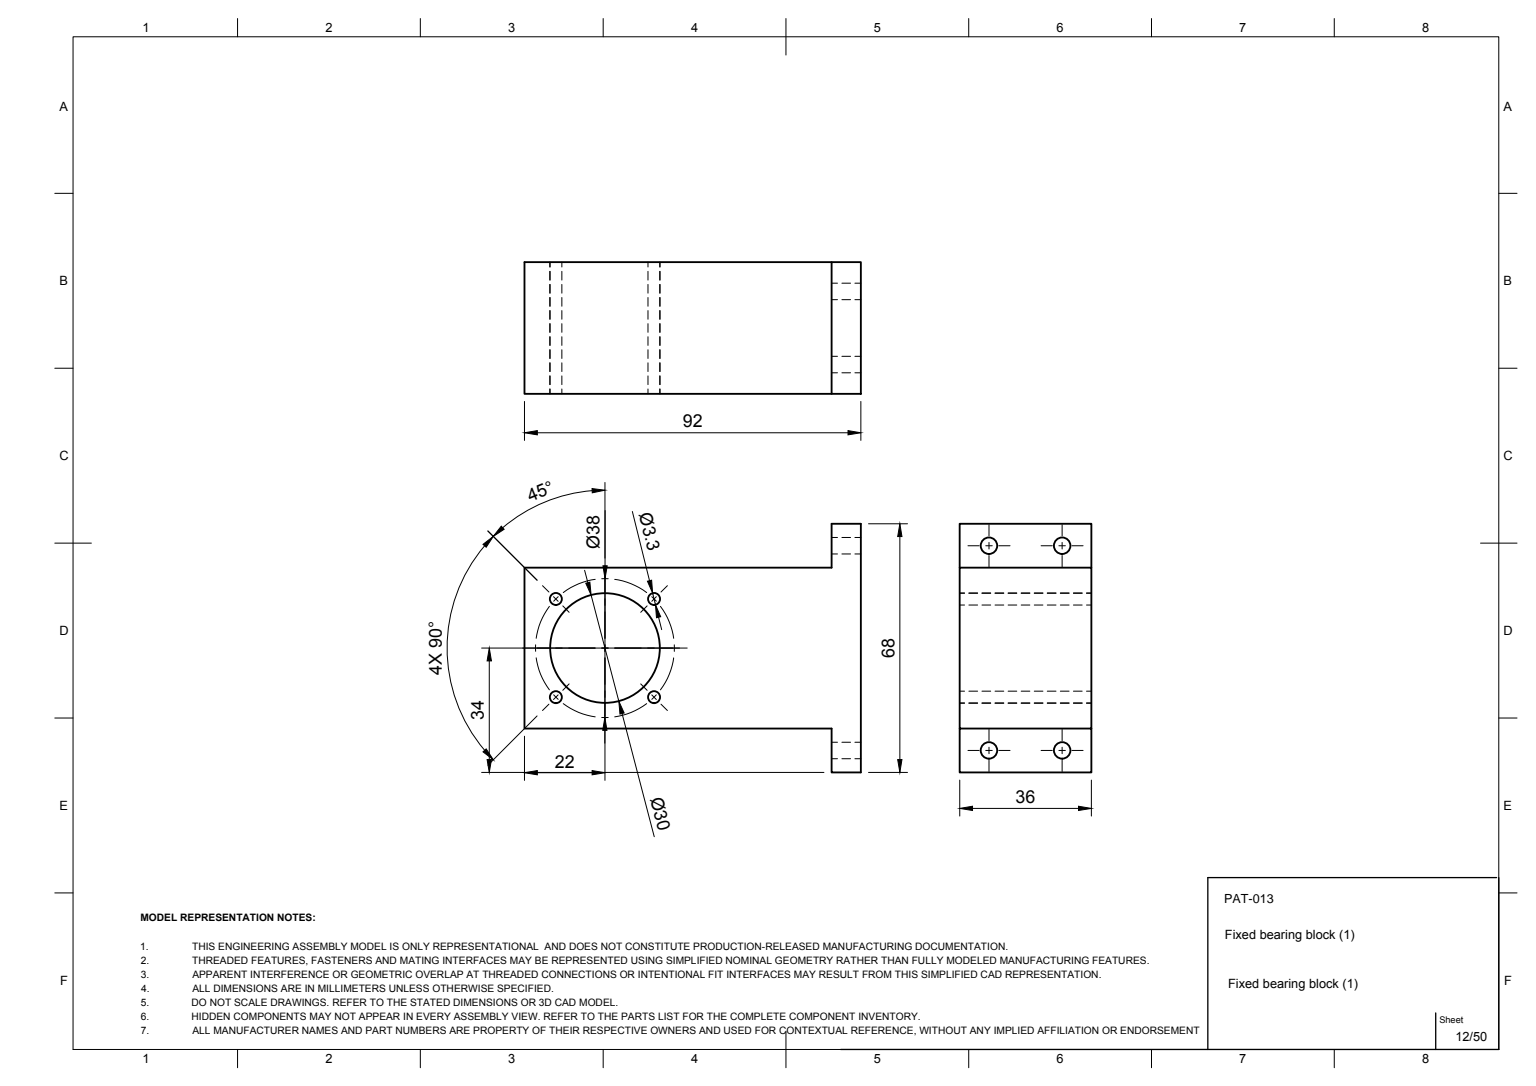
ISO-10303-21;
HEADER;
/* Generated by software containing ST-Developer
 * from STEP Tools, Inc. (www.steptools.com) 
 */

FILE_DESCRIPTION(
/* description */ ('Belt-driven linear axis on 2020 extrusion'),
/* implementation_level */ '2;1');

FILE_NAME(
/* name */ 'Fixed bearing block (1).step',
/* time_stamp */ '2026-10-28T03:26:09-07:00',
/* author */ (''),
/* organization */ (''),
/* preprocessor_version */ 'ST-DEVELOPER v20.2',
/* originating_system */ 'Autodesk Translation Framework v15.17.0.0',
/* authorisation */ '');

FILE_SCHEMA (('AUTOMOTIVE_DESIGN { 1 0 10303 214 3 1 1 }'));
ENDSEC;

DATA;
#10=MECHANICAL_DESIGN_GEOMETRIC_PRESENTATION_REPRESENTATION('',(#619),#20096);
#525=SHAPE_REPRESENTATION_RELATIONSHIP('SRR','None',#20321,#571);
#571=ADVANCED_BREP_SHAPE_REPRESENTATION('',(#675),#20052);
#619=STYLED_ITEM('',(#20650),#675);
#675=MANIFOLD_SOLID_BREP('Body1',#10932);
#768=FACE_BOUND('',#2047,.T.);
#769=FACE_BOUND('',#2048,.T.);
#770=FACE_BOUND('',#2050,.T.);
#771=FACE_BOUND('',#2051,.T.);
#772=FACE_BOUND('',#2055,.T.);
#773=FACE_BOUND('',#2056,.T.);
#774=FACE_BOUND('',#2057,.T.);
#775=FACE_BOUND('',#2058,.T.);
#776=FACE_BOUND('',#2059,.T.);
#777=FACE_BOUND('',#2062,.T.);
#778=FACE_BOUND('',#2063,.T.);
#779=FACE_BOUND('',#2064,.T.);
#780=FACE_BOUND('',#2065,.T.);
#781=FACE_BOUND('',#2066,.T.);
#782=FACE_BOUND('',#2070,.T.);
#783=FACE_BOUND('',#2071,.T.);
#784=FACE_BOUND('',#2072,.T.);
#785=FACE_BOUND('',#2073,.T.);
#953=PLANE('',#11744);
#954=PLANE('',#11745);
#955=PLANE('',#11746);
#956=PLANE('',#11747);
#957=PLANE('',#11748);
#958=PLANE('',#11749);
#959=PLANE('',#11750);
#960=PLANE('',#11751);
#961=PLANE('',#11752);
#962=PLANE('',#11753);
#1365=FACE_OUTER_BOUND('',#2037,.T.);
#1366=FACE_OUTER_BOUND('',#2038,.T.);
#1367=FACE_OUTER_BOUND('',#2039,.T.);
#1368=FACE_OUTER_BOUND('',#2040,.T.);
#1369=FACE_OUTER_BOUND('',#2041,.T.);
#1370=FACE_OUTER_BOUND('',#2042,.T.);
#1371=FACE_OUTER_BOUND('',#2043,.T.);
#1372=FACE_OUTER_BOUND('',#2044,.T.);
#1373=FACE_OUTER_BOUND('',#2045,.T.);
#1374=FACE_OUTER_BOUND('',#2046,.T.);
#1375=FACE_OUTER_BOUND('',#2049,.T.);
#1376=FACE_OUTER_BOUND('',#2052,.T.);
#1377=FACE_OUTER_BOUND('',#2053,.T.);
#1378=FACE_OUTER_BOUND('',#2054,.T.);
#1379=FACE_OUTER_BOUND('',#2060,.T.);
#1380=FACE_OUTER_BOUND('',#2061,.T.);
#1381=FACE_OUTER_BOUND('',#2067,.T.);
#1382=FACE_OUTER_BOUND('',#2068,.T.);
#1383=FACE_OUTER_BOUND('',#2069,.T.);
#2037=EDGE_LOOP('',(#7727,#7728,#7729,#7730));
#2038=EDGE_LOOP('',(#7731,#7732,#7733,#7734));
#2039=EDGE_LOOP('',(#7735,#7736,#7737,#7738));
#2040=EDGE_LOOP('',(#7739,#7740,#7741,#7742));
#2041=EDGE_LOOP('',(#7743,#7744,#7745,#7746));
#2042=EDGE_LOOP('',(#7747,#7748,#7749,#7750));
#2043=EDGE_LOOP('',(#7751,#7752,#7753,#7754));
#2044=EDGE_LOOP('',(#7755,#7756,#7757,#7758));
#2045=EDGE_LOOP('',(#7759,#7760,#7761,#7762));
#2046=EDGE_LOOP('',(#7763,#7764,#7765,#7766));
#2047=EDGE_LOOP('',(#7767));
#2048=EDGE_LOOP('',(#7768));
#2049=EDGE_LOOP('',(#7769,#7770,#7771,#7772));
#2050=EDGE_LOOP('',(#7773));
#2051=EDGE_LOOP('',(#7774));
#2052=EDGE_LOOP('',(#7775,#7776,#7777,#7778));
#2053=EDGE_LOOP('',(#7779,#7780,#7781,#7782));
#2054=EDGE_LOOP('',(#7783,#7784,#7785,#7786,#7787,#7788,#7789,#7790));
#2055=EDGE_LOOP('',(#7791));
#2056=EDGE_LOOP('',(#7792));
#2057=EDGE_LOOP('',(#7793));
#2058=EDGE_LOOP('',(#7794));
#2059=EDGE_LOOP('',(#7795));
#2060=EDGE_LOOP('',(#7796,#7797,#7798,#7799));
#2061=EDGE_LOOP('',(#7800,#7801,#7802,#7803,#7804,#7805,#7806,#7807));
#2062=EDGE_LOOP('',(#7808));
#2063=EDGE_LOOP('',(#7809));
#2064=EDGE_LOOP('',(#7810));
#2065=EDGE_LOOP('',(#7811));
#2066=EDGE_LOOP('',(#7812));
#2067=EDGE_LOOP('',(#7813,#7814,#7815,#7816));
#2068=EDGE_LOOP('',(#7817,#7818,#7819,#7820));
#2069=EDGE_LOOP('',(#7821,#7822,#7823,#7824));
#2070=EDGE_LOOP('',(#7825));
#2071=EDGE_LOOP('',(#7826));
#2072=EDGE_LOOP('',(#7827));
#2073=EDGE_LOOP('',(#7828));
#2800=LINE('',#16756,#3657);
#2801=LINE('',#16762,#3658);
#2802=LINE('',#16768,#3659);
#2803=LINE('',#16774,#3660);
#2804=LINE('',#16780,#3661);
#2805=LINE('',#16786,#3662);
#2806=LINE('',#16792,#3663);
#2807=LINE('',#16798,#3664);
#2808=LINE('',#16804,#3665);
#2809=LINE('',#16809,#3666);
#2810=LINE('',#16811,#3667);
#2811=LINE('',#16813,#3668);
#2812=LINE('',#16814,#3669);
#2813=LINE('',#16818,#3670);
#2814=LINE('',#16820,#3671);
#2815=LINE('',#16822,#3672);
#2816=LINE('',#16823,#3673);
#2817=LINE('',#16826,#3674);
#2818=LINE('',#16828,#3675);
#2819=LINE('',#16829,#3676);
#2820=LINE('',#16832,#3677);
#2821=LINE('',#16834,#3678);
#2822=LINE('',#16835,#3679);
#2823=LINE('',#16838,#3680);
#2824=LINE('',#16840,#3681);
#2825=LINE('',#16841,#3682);
#2826=LINE('',#16842,#3683);
#2827=LINE('',#16845,#3684);
#2828=LINE('',#16846,#3685);
#2829=LINE('',#16849,#3686);
#2830=LINE('',#16850,#3687);
#2831=LINE('',#16851,#3688);
#2832=LINE('',#16853,#3689);
#3657=VECTOR('',#13378,0.164999999999999);
#3658=VECTOR('',#13385,0.164999999999999);
#3659=VECTOR('',#13392,0.164999999999999);
#3660=VECTOR('',#13399,0.164999999999999);
#3661=VECTOR('',#13406,1.5);
#3662=VECTOR('',#13413,0.225000000000001);
#3663=VECTOR('',#13420,0.225000000000001);
#3664=VECTOR('',#13427,0.225000000000001);
#3665=VECTOR('',#13434,0.225000000000001);
#3666=VECTOR('',#13439,1.);
#3667=VECTOR('',#13440,1.);
#3668=VECTOR('',#13441,1.);
#3669=VECTOR('',#13442,1.);
#3670=VECTOR('',#13445,1.);
#3671=VECTOR('',#13446,1.);
#3672=VECTOR('',#13447,1.);
#3673=VECTOR('',#13448,1.);
#3674=VECTOR('',#13451,1.);
#3675=VECTOR('',#13452,1.);
#3676=VECTOR('',#13453,1.);
#3677=VECTOR('',#13456,1.);
#3678=VECTOR('',#13457,1.);
#3679=VECTOR('',#13458,1.);
#3680=VECTOR('',#13461,1.);
#3681=VECTOR('',#13462,1.);
#3682=VECTOR('',#13463,1.);
#3683=VECTOR('',#13464,1.);
#3684=VECTOR('',#13467,1.);
#3685=VECTOR('',#13468,1.);
#3686=VECTOR('',#13471,1.);
#3687=VECTOR('',#13472,1.);
#3688=VECTOR('',#13473,1.);
#3689=VECTOR('',#13476,1.);
#4481=CIRCLE('',#11718,0.164999999999999);
#4482=CIRCLE('',#11719,0.164999999999999);
#4483=CIRCLE('',#11721,0.164999999999999);
#4484=CIRCLE('',#11722,0.164999999999999);
#4485=CIRCLE('',#11724,0.164999999999999);
#4486=CIRCLE('',#11725,0.164999999999999);
#4487=CIRCLE('',#11727,0.164999999999999);
#4488=CIRCLE('',#11728,0.164999999999999);
#4489=CIRCLE('',#11730,1.5);
#4490=CIRCLE('',#11731,1.5);
#4491=CIRCLE('',#11733,0.225000000000001);
#4492=CIRCLE('',#11734,0.225000000000001);
#4493=CIRCLE('',#11736,0.225000000000001);
#4494=CIRCLE('',#11737,0.225000000000001);
#4495=CIRCLE('',#11739,0.225000000000001);
#4496=CIRCLE('',#11740,0.225000000000001);
#4497=CIRCLE('',#11742,0.225000000000001);
#4498=CIRCLE('',#11743,0.225000000000001);
#5050=VERTEX_POINT('',#16753);
#5051=VERTEX_POINT('',#16755);
#5052=VERTEX_POINT('',#16759);
#5053=VERTEX_POINT('',#16761);
#5054=VERTEX_POINT('',#16765);
#5055=VERTEX_POINT('',#16767);
#5056=VERTEX_POINT('',#16771);
#5057=VERTEX_POINT('',#16773);
#5058=VERTEX_POINT('',#16777);
#5059=VERTEX_POINT('',#16779);
#5060=VERTEX_POINT('',#16783);
#5061=VERTEX_POINT('',#16785);
#5062=VERTEX_POINT('',#16789);
#5063=VERTEX_POINT('',#16791);
#5064=VERTEX_POINT('',#16795);
#5065=VERTEX_POINT('',#16797);
#5066=VERTEX_POINT('',#16801);
#5067=VERTEX_POINT('',#16803);
#5068=VERTEX_POINT('',#16807);
#5069=VERTEX_POINT('',#16808);
#5070=VERTEX_POINT('',#16810);
#5071=VERTEX_POINT('',#16812);
#5072=VERTEX_POINT('',#16816);
#5073=VERTEX_POINT('',#16817);
#5074=VERTEX_POINT('',#16819);
#5075=VERTEX_POINT('',#16821);
#5076=VERTEX_POINT('',#16825);
#5077=VERTEX_POINT('',#16827);
#5078=VERTEX_POINT('',#16831);
#5079=VERTEX_POINT('',#16833);
#5080=VERTEX_POINT('',#16837);
#5081=VERTEX_POINT('',#16839);
#5082=VERTEX_POINT('',#16844);
#5083=VERTEX_POINT('',#16848);
#6078=EDGE_CURVE('',#5050,#5050,#4481,.T.);
#6079=EDGE_CURVE('',#5050,#5051,#2800,.T.);
#6080=EDGE_CURVE('',#5051,#5051,#4482,.T.);
#6081=EDGE_CURVE('',#5052,#5052,#4483,.T.);
#6082=EDGE_CURVE('',#5052,#5053,#2801,.T.);
#6083=EDGE_CURVE('',#5053,#5053,#4484,.T.);
#6084=EDGE_CURVE('',#5054,#5054,#4485,.T.);
#6085=EDGE_CURVE('',#5054,#5055,#2802,.T.);
#6086=EDGE_CURVE('',#5055,#5055,#4486,.T.);
#6087=EDGE_CURVE('',#5056,#5056,#4487,.T.);
#6088=EDGE_CURVE('',#5056,#5057,#2803,.T.);
#6089=EDGE_CURVE('',#5057,#5057,#4488,.T.);
#6090=EDGE_CURVE('',#5058,#5058,#4489,.T.);
#6091=EDGE_CURVE('',#5058,#5059,#2804,.T.);
#6092=EDGE_CURVE('',#5059,#5059,#4490,.T.);
#6093=EDGE_CURVE('',#5060,#5060,#4491,.T.);
#6094=EDGE_CURVE('',#5060,#5061,#2805,.T.);
#6095=EDGE_CURVE('',#5061,#5061,#4492,.T.);
#6096=EDGE_CURVE('',#5062,#5062,#4493,.T.);
#6097=EDGE_CURVE('',#5062,#5063,#2806,.T.);
#6098=EDGE_CURVE('',#5063,#5063,#4494,.T.);
#6099=EDGE_CURVE('',#5064,#5064,#4495,.T.);
#6100=EDGE_CURVE('',#5064,#5065,#2807,.T.);
#6101=EDGE_CURVE('',#5065,#5065,#4496,.T.);
#6102=EDGE_CURVE('',#5066,#5066,#4497,.T.);
#6103=EDGE_CURVE('',#5066,#5067,#2808,.T.);
#6104=EDGE_CURVE('',#5067,#5067,#4498,.T.);
#6105=EDGE_CURVE('',#5068,#5069,#2809,.T.);
#6106=EDGE_CURVE('',#5070,#5068,#2810,.T.);
#6107=EDGE_CURVE('',#5070,#5071,#2811,.T.);
#6108=EDGE_CURVE('',#5069,#5071,#2812,.T.);
#6109=EDGE_CURVE('',#5072,#5073,#2813,.T.);
#6110=EDGE_CURVE('',#5074,#5072,#2814,.T.);
#6111=EDGE_CURVE('',#5075,#5074,#2815,.T.);
#6112=EDGE_CURVE('',#5073,#5075,#2816,.T.);
#6113=EDGE_CURVE('',#5075,#5076,#2817,.T.);
#6114=EDGE_CURVE('',#5077,#5074,#2818,.T.);
#6115=EDGE_CURVE('',#5076,#5077,#2819,.T.);
#6116=EDGE_CURVE('',#5078,#5070,#2820,.T.);
#6117=EDGE_CURVE('',#5078,#5079,#2821,.T.);
#6118=EDGE_CURVE('',#5071,#5079,#2822,.T.);
#6119=EDGE_CURVE('',#5068,#5080,#2823,.T.);
#6120=EDGE_CURVE('',#5081,#5080,#2824,.T.);
#6121=EDGE_CURVE('',#5073,#5081,#2825,.T.);
#6122=EDGE_CURVE('',#5076,#5078,#2826,.T.);
#6123=EDGE_CURVE('',#5069,#5082,#2827,.T.);
#6124=EDGE_CURVE('',#5080,#5082,#2828,.T.);
#6125=EDGE_CURVE('',#5072,#5083,#2829,.T.);
#6126=EDGE_CURVE('',#5082,#5083,#2830,.T.);
#6127=EDGE_CURVE('',#5079,#5077,#2831,.T.);
#6128=EDGE_CURVE('',#5083,#5081,#2832,.T.);
#7727=ORIENTED_EDGE('',*,*,#6078,.F.);
#7728=ORIENTED_EDGE('',*,*,#6079,.T.);
#7729=ORIENTED_EDGE('',*,*,#6080,.F.);
#7730=ORIENTED_EDGE('',*,*,#6079,.F.);
#7731=ORIENTED_EDGE('',*,*,#6081,.F.);
#7732=ORIENTED_EDGE('',*,*,#6082,.T.);
#7733=ORIENTED_EDGE('',*,*,#6083,.F.);
#7734=ORIENTED_EDGE('',*,*,#6082,.F.);
#7735=ORIENTED_EDGE('',*,*,#6084,.F.);
#7736=ORIENTED_EDGE('',*,*,#6085,.T.);
#7737=ORIENTED_EDGE('',*,*,#6086,.F.);
#7738=ORIENTED_EDGE('',*,*,#6085,.F.);
#7739=ORIENTED_EDGE('',*,*,#6087,.F.);
#7740=ORIENTED_EDGE('',*,*,#6088,.T.);
#7741=ORIENTED_EDGE('',*,*,#6089,.F.);
#7742=ORIENTED_EDGE('',*,*,#6088,.F.);
#7743=ORIENTED_EDGE('',*,*,#6090,.F.);
#7744=ORIENTED_EDGE('',*,*,#6091,.T.);
#7745=ORIENTED_EDGE('',*,*,#6092,.F.);
#7746=ORIENTED_EDGE('',*,*,#6091,.F.);
#7747=ORIENTED_EDGE('',*,*,#6093,.F.);
#7748=ORIENTED_EDGE('',*,*,#6094,.T.);
#7749=ORIENTED_EDGE('',*,*,#6095,.F.);
#7750=ORIENTED_EDGE('',*,*,#6094,.F.);
#7751=ORIENTED_EDGE('',*,*,#6096,.F.);
#7752=ORIENTED_EDGE('',*,*,#6097,.T.);
#7753=ORIENTED_EDGE('',*,*,#6098,.F.);
#7754=ORIENTED_EDGE('',*,*,#6097,.F.);
#7755=ORIENTED_EDGE('',*,*,#6099,.F.);
#7756=ORIENTED_EDGE('',*,*,#6100,.T.);
#7757=ORIENTED_EDGE('',*,*,#6101,.F.);
#7758=ORIENTED_EDGE('',*,*,#6100,.F.);
#7759=ORIENTED_EDGE('',*,*,#6102,.F.);
#7760=ORIENTED_EDGE('',*,*,#6103,.T.);
#7761=ORIENTED_EDGE('',*,*,#6104,.F.);
#7762=ORIENTED_EDGE('',*,*,#6103,.F.);
#7763=ORIENTED_EDGE('',*,*,#6105,.F.);
#7764=ORIENTED_EDGE('',*,*,#6106,.F.);
#7765=ORIENTED_EDGE('',*,*,#6107,.T.);
#7766=ORIENTED_EDGE('',*,*,#6108,.F.);
#7767=ORIENTED_EDGE('',*,*,#6095,.T.);
#7768=ORIENTED_EDGE('',*,*,#6104,.T.);
#7769=ORIENTED_EDGE('',*,*,#6109,.F.);
#7770=ORIENTED_EDGE('',*,*,#6110,.F.);
#7771=ORIENTED_EDGE('',*,*,#6111,.F.);
#7772=ORIENTED_EDGE('',*,*,#6112,.F.);
#7773=ORIENTED_EDGE('',*,*,#6098,.T.);
#7774=ORIENTED_EDGE('',*,*,#6101,.T.);
#7775=ORIENTED_EDGE('',*,*,#6113,.F.);
#7776=ORIENTED_EDGE('',*,*,#6111,.T.);
#7777=ORIENTED_EDGE('',*,*,#6114,.F.);
#7778=ORIENTED_EDGE('',*,*,#6115,.F.);
#7779=ORIENTED_EDGE('',*,*,#6116,.F.);
#7780=ORIENTED_EDGE('',*,*,#6117,.T.);
#7781=ORIENTED_EDGE('',*,*,#6118,.F.);
#7782=ORIENTED_EDGE('',*,*,#6107,.F.);
#7783=ORIENTED_EDGE('',*,*,#6119,.T.);
#7784=ORIENTED_EDGE('',*,*,#6120,.F.);
#7785=ORIENTED_EDGE('',*,*,#6121,.F.);
#7786=ORIENTED_EDGE('',*,*,#6112,.T.);
#7787=ORIENTED_EDGE('',*,*,#6113,.T.);
#7788=ORIENTED_EDGE('',*,*,#6122,.T.);
#7789=ORIENTED_EDGE('',*,*,#6116,.T.);
#7790=ORIENTED_EDGE('',*,*,#6106,.T.);
#7791=ORIENTED_EDGE('',*,*,#6090,.T.);
#7792=ORIENTED_EDGE('',*,*,#6087,.T.);
#7793=ORIENTED_EDGE('',*,*,#6084,.T.);
#7794=ORIENTED_EDGE('',*,*,#6081,.T.);
#7795=ORIENTED_EDGE('',*,*,#6078,.T.);
#7796=ORIENTED_EDGE('',*,*,#6105,.T.);
#7797=ORIENTED_EDGE('',*,*,#6123,.T.);
#7798=ORIENTED_EDGE('',*,*,#6124,.F.);
#7799=ORIENTED_EDGE('',*,*,#6119,.F.);
#7800=ORIENTED_EDGE('',*,*,#6125,.T.);
#7801=ORIENTED_EDGE('',*,*,#6126,.F.);
#7802=ORIENTED_EDGE('',*,*,#6123,.F.);
#7803=ORIENTED_EDGE('',*,*,#6108,.T.);
#7804=ORIENTED_EDGE('',*,*,#6118,.T.);
#7805=ORIENTED_EDGE('',*,*,#6127,.T.);
#7806=ORIENTED_EDGE('',*,*,#6114,.T.);
#7807=ORIENTED_EDGE('',*,*,#6110,.T.);
#7808=ORIENTED_EDGE('',*,*,#6092,.T.);
#7809=ORIENTED_EDGE('',*,*,#6089,.T.);
#7810=ORIENTED_EDGE('',*,*,#6086,.T.);
#7811=ORIENTED_EDGE('',*,*,#6083,.T.);
#7812=ORIENTED_EDGE('',*,*,#6080,.T.);
#7813=ORIENTED_EDGE('',*,*,#6109,.T.);
#7814=ORIENTED_EDGE('',*,*,#6121,.T.);
#7815=ORIENTED_EDGE('',*,*,#6128,.F.);
#7816=ORIENTED_EDGE('',*,*,#6125,.F.);
#7817=ORIENTED_EDGE('',*,*,#6128,.T.);
#7818=ORIENTED_EDGE('',*,*,#6120,.T.);
#7819=ORIENTED_EDGE('',*,*,#6124,.T.);
#7820=ORIENTED_EDGE('',*,*,#6126,.T.);
#7821=ORIENTED_EDGE('',*,*,#6127,.F.);
#7822=ORIENTED_EDGE('',*,*,#6117,.F.);
#7823=ORIENTED_EDGE('',*,*,#6122,.F.);
#7824=ORIENTED_EDGE('',*,*,#6115,.T.);
#7825=ORIENTED_EDGE('',*,*,#6093,.T.);
#7826=ORIENTED_EDGE('',*,*,#6096,.T.);
#7827=ORIENTED_EDGE('',*,*,#6099,.T.);
#7828=ORIENTED_EDGE('',*,*,#6102,.T.);
#10128=CYLINDRICAL_SURFACE('',#11717,0.164999999999999);
#10129=CYLINDRICAL_SURFACE('',#11720,0.164999999999999);
#10130=CYLINDRICAL_SURFACE('',#11723,0.164999999999999);
#10131=CYLINDRICAL_SURFACE('',#11726,0.164999999999999);
#10132=CYLINDRICAL_SURFACE('',#11729,1.5);
#10133=CYLINDRICAL_SURFACE('',#11732,0.225000000000001);
#10134=CYLINDRICAL_SURFACE('',#11735,0.225000000000001);
#10135=CYLINDRICAL_SURFACE('',#11738,0.225000000000001);
#10136=CYLINDRICAL_SURFACE('',#11741,0.225000000000001);
#10416=ADVANCED_FACE('',(#1365),#10128,.F.);
#10417=ADVANCED_FACE('',(#1366),#10129,.F.);
#10418=ADVANCED_FACE('',(#1367),#10130,.F.);
#10419=ADVANCED_FACE('',(#1368),#10131,.F.);
#10420=ADVANCED_FACE('',(#1369),#10132,.F.);
#10421=ADVANCED_FACE('',(#1370),#10133,.F.);
#10422=ADVANCED_FACE('',(#1371),#10134,.F.);
#10423=ADVANCED_FACE('',(#1372),#10135,.F.);
#10424=ADVANCED_FACE('',(#1373),#10136,.F.);
#10425=ADVANCED_FACE('',(#1374,#768,#769),#953,.T.);
#10426=ADVANCED_FACE('',(#1375,#770,#771),#954,.T.);
#10427=ADVANCED_FACE('',(#1376),#955,.T.);
#10428=ADVANCED_FACE('',(#1377),#956,.T.);
#10429=ADVANCED_FACE('',(#1378,#772,#773,#774,#775,#776),#957,.T.);
#10430=ADVANCED_FACE('',(#1379),#958,.T.);
#10431=ADVANCED_FACE('',(#1380,#777,#778,#779,#780,#781),#959,.T.);
#10432=ADVANCED_FACE('',(#1381),#960,.T.);
#10433=ADVANCED_FACE('',(#1382),#961,.T.);
#10434=ADVANCED_FACE('',(#1383,#782,#783,#784,#785),#962,.F.);
#10932=CLOSED_SHELL('',(#10416,#10417,#10418,#10419,#10420,#10421,#10422,
#10423,#10424,#10425,#10426,#10427,#10428,#10429,#10430,#10431,#10432,#10433,
#10434));
#11716=AXIS2_PLACEMENT_3D('',#16751,#13372,#13373);
#11717=AXIS2_PLACEMENT_3D('',#16752,#13374,#13375);
#11718=AXIS2_PLACEMENT_3D('',#16754,#13376,#13377);
#11719=AXIS2_PLACEMENT_3D('',#16757,#13379,#13380);
#11720=AXIS2_PLACEMENT_3D('',#16758,#13381,#13382);
#11721=AXIS2_PLACEMENT_3D('',#16760,#13383,#13384);
#11722=AXIS2_PLACEMENT_3D('',#16763,#13386,#13387);
#11723=AXIS2_PLACEMENT_3D('',#16764,#13388,#13389);
#11724=AXIS2_PLACEMENT_3D('',#16766,#13390,#13391);
#11725=AXIS2_PLACEMENT_3D('',#16769,#13393,#13394);
#11726=AXIS2_PLACEMENT_3D('',#16770,#13395,#13396);
#11727=AXIS2_PLACEMENT_3D('',#16772,#13397,#13398);
#11728=AXIS2_PLACEMENT_3D('',#16775,#13400,#13401);
#11729=AXIS2_PLACEMENT_3D('',#16776,#13402,#13403);
#11730=AXIS2_PLACEMENT_3D('',#16778,#13404,#13405);
#11731=AXIS2_PLACEMENT_3D('',#16781,#13407,#13408);
#11732=AXIS2_PLACEMENT_3D('',#16782,#13409,#13410);
#11733=AXIS2_PLACEMENT_3D('',#16784,#13411,#13412);
#11734=AXIS2_PLACEMENT_3D('',#16787,#13414,#13415);
#11735=AXIS2_PLACEMENT_3D('',#16788,#13416,#13417);
#11736=AXIS2_PLACEMENT_3D('',#16790,#13418,#13419);
#11737=AXIS2_PLACEMENT_3D('',#16793,#13421,#13422);
#11738=AXIS2_PLACEMENT_3D('',#16794,#13423,#13424);
#11739=AXIS2_PLACEMENT_3D('',#16796,#13425,#13426);
#11740=AXIS2_PLACEMENT_3D('',#16799,#13428,#13429);
#11741=AXIS2_PLACEMENT_3D('',#16800,#13430,#13431);
#11742=AXIS2_PLACEMENT_3D('',#16802,#13432,#13433);
#11743=AXIS2_PLACEMENT_3D('',#16805,#13435,#13436);
#11744=AXIS2_PLACEMENT_3D('',#16806,#13437,#13438);
#11745=AXIS2_PLACEMENT_3D('',#16815,#13443,#13444);
#11746=AXIS2_PLACEMENT_3D('',#16824,#13449,#13450);
#11747=AXIS2_PLACEMENT_3D('',#16830,#13454,#13455);
#11748=AXIS2_PLACEMENT_3D('',#16836,#13459,#13460);
#11749=AXIS2_PLACEMENT_3D('',#16843,#13465,#13466);
#11750=AXIS2_PLACEMENT_3D('',#16847,#13469,#13470);
#11751=AXIS2_PLACEMENT_3D('',#16852,#13474,#13475);
#11752=AXIS2_PLACEMENT_3D('',#16854,#13477,#13478);
#11753=AXIS2_PLACEMENT_3D('',#16855,#13479,#13480);
#13372=DIRECTION('axis',(0.,0.,1.));
#13373=DIRECTION('refdir',(1.,0.,0.));
#13374=DIRECTION('center_axis',(0.,1.,0.));
#13375=DIRECTION('ref_axis',(1.,0.,0.));
#13376=DIRECTION('center_axis',(0.,1.,0.));
#13377=DIRECTION('ref_axis',(1.,0.,0.));
#13378=DIRECTION('',(0.,1.,0.));
#13379=DIRECTION('center_axis',(0.,-1.,0.));
#13380=DIRECTION('ref_axis',(1.,0.,0.));
#13381=DIRECTION('center_axis',(0.,1.,0.));
#13382=DIRECTION('ref_axis',(1.,0.,0.));
#13383=DIRECTION('center_axis',(0.,1.,0.));
#13384=DIRECTION('ref_axis',(1.,0.,0.));
#13385=DIRECTION('',(0.,1.,0.));
#13386=DIRECTION('center_axis',(0.,-1.,0.));
#13387=DIRECTION('ref_axis',(1.,0.,0.));
#13388=DIRECTION('center_axis',(0.,1.,0.));
#13389=DIRECTION('ref_axis',(1.,0.,0.));
#13390=DIRECTION('center_axis',(0.,1.,0.));
#13391=DIRECTION('ref_axis',(1.,0.,0.));
#13392=DIRECTION('',(0.,1.,0.));
#13393=DIRECTION('center_axis',(0.,-1.,0.));
#13394=DIRECTION('ref_axis',(1.,0.,0.));
#13395=DIRECTION('center_axis',(0.,1.,0.));
#13396=DIRECTION('ref_axis',(1.,0.,0.));
#13397=DIRECTION('center_axis',(0.,1.,0.));
#13398=DIRECTION('ref_axis',(1.,0.,0.));
#13399=DIRECTION('',(0.,1.,0.));
#13400=DIRECTION('center_axis',(0.,-1.,0.));
#13401=DIRECTION('ref_axis',(1.,0.,0.));
#13402=DIRECTION('center_axis',(0.,1.,0.));
#13403=DIRECTION('ref_axis',(1.,0.,0.));
#13404=DIRECTION('center_axis',(0.,1.,0.));
#13405=DIRECTION('ref_axis',(1.,0.,0.));
#13406=DIRECTION('',(0.,1.,0.));
#13407=DIRECTION('center_axis',(0.,-1.,0.));
#13408=DIRECTION('ref_axis',(1.,0.,0.));
#13409=DIRECTION('center_axis',(0.,0.,1.));
#13410=DIRECTION('ref_axis',(1.,0.,0.));
#13411=DIRECTION('center_axis',(0.,0.,1.));
#13412=DIRECTION('ref_axis',(1.,0.,0.));
#13413=DIRECTION('',(0.,0.,1.));
#13414=DIRECTION('center_axis',(0.,0.,-1.));
#13415=DIRECTION('ref_axis',(1.,0.,0.));
#13416=DIRECTION('center_axis',(0.,0.,1.));
#13417=DIRECTION('ref_axis',(1.,0.,0.));
#13418=DIRECTION('center_axis',(0.,0.,1.));
#13419=DIRECTION('ref_axis',(1.,0.,0.));
#13420=DIRECTION('',(0.,0.,1.));
#13421=DIRECTION('center_axis',(0.,0.,-1.));
#13422=DIRECTION('ref_axis',(1.,0.,0.));
#13423=DIRECTION('center_axis',(0.,0.,1.));
#13424=DIRECTION('ref_axis',(1.,0.,0.));
#13425=DIRECTION('center_axis',(0.,0.,1.));
#13426=DIRECTION('ref_axis',(1.,0.,0.));
#13427=DIRECTION('',(0.,0.,1.));
#13428=DIRECTION('center_axis',(0.,0.,-1.));
#13429=DIRECTION('ref_axis',(1.,0.,0.));
#13430=DIRECTION('center_axis',(0.,0.,1.));
#13431=DIRECTION('ref_axis',(1.,0.,0.));
#13432=DIRECTION('center_axis',(0.,0.,1.));
#13433=DIRECTION('ref_axis',(1.,0.,0.));
#13434=DIRECTION('',(0.,0.,1.));
#13435=DIRECTION('center_axis',(0.,0.,-1.));
#13436=DIRECTION('ref_axis',(1.,0.,0.));
#13437=DIRECTION('center_axis',(0.,0.,1.));
#13438=DIRECTION('ref_axis',(1.,0.,0.));
#13439=DIRECTION('',(0.,1.,0.));
#13440=DIRECTION('',(-1.,0.,0.));
#13441=DIRECTION('',(0.,1.,0.));
#13442=DIRECTION('',(1.,0.,0.));
#13443=DIRECTION('center_axis',(0.,0.,1.));
#13444=DIRECTION('ref_axis',(1.,0.,0.));
#13445=DIRECTION('',(0.,-1.,0.));
#13446=DIRECTION('',(1.,0.,0.));
#13447=DIRECTION('',(0.,1.,0.));
#13448=DIRECTION('',(-1.,0.,0.));
#13449=DIRECTION('center_axis',(-1.,0.,0.));
#13450=DIRECTION('ref_axis',(0.,0.,1.));
#13451=DIRECTION('',(0.,0.,-1.));
#13452=DIRECTION('',(0.,0.,1.));
#13453=DIRECTION('',(0.,1.,0.));
#13454=DIRECTION('center_axis',(1.,0.,0.));
#13455=DIRECTION('ref_axis',(0.,0.,-1.));
#13456=DIRECTION('',(0.,0.,1.));
#13457=DIRECTION('',(0.,1.,0.));
#13458=DIRECTION('',(0.,0.,-1.));
#13459=DIRECTION('center_axis',(0.,-1.,0.));
#13460=DIRECTION('ref_axis',(1.,0.,0.));
#13461=DIRECTION('',(0.,0.,1.));
#13462=DIRECTION('',(1.,0.,0.));
#13463=DIRECTION('',(0.,0.,1.));
#13464=DIRECTION('',(1.,0.,0.));
#13465=DIRECTION('center_axis',(1.,0.,0.));
#13466=DIRECTION('ref_axis',(0.,1.,0.));
#13467=DIRECTION('',(0.,0.,1.));
#13468=DIRECTION('',(0.,1.,0.));
#13469=DIRECTION('center_axis',(0.,1.,0.));
#13470=DIRECTION('ref_axis',(-1.,0.,0.));
#13471=DIRECTION('',(0.,0.,1.));
#13472=DIRECTION('',(-1.,0.,0.));
#13473=DIRECTION('',(-1.,0.,0.));
#13474=DIRECTION('center_axis',(-1.,0.,0.));
#13475=DIRECTION('ref_axis',(0.,-1.,0.));
#13476=DIRECTION('',(0.,-1.,0.));
#13477=DIRECTION('center_axis',(0.,0.,1.));
#13478=DIRECTION('ref_axis',(1.,0.,0.));
#13479=DIRECTION('center_axis',(0.,0.,1.));
#13480=DIRECTION('ref_axis',(1.,0.,0.));
#16751=CARTESIAN_POINT('',(0.,0.,0.));
#16752=CARTESIAN_POINT('Origin',(30.6564971157456,-1.9,5.65649711574556));
#16753=CARTESIAN_POINT('',(30.4914971157456,-1.8,5.65649711574556));
#16754=CARTESIAN_POINT('Origin',(30.6564971157456,-1.8,5.65649711574556));
#16755=CARTESIAN_POINT('',(30.4914971157456,1.8,5.65649711574556));
#16756=CARTESIAN_POINT('',(30.4914971157456,-1.9,5.65649711574556));
#16757=CARTESIAN_POINT('Origin',(30.6564971157456,1.8,5.65649711574556));
#16758=CARTESIAN_POINT('Origin',(30.6564971157456,-1.9,8.34350288425444));
#16759=CARTESIAN_POINT('',(30.4914971157456,-1.8,8.34350288425444));
#16760=CARTESIAN_POINT('Origin',(30.6564971157456,-1.8,8.34350288425444));
#16761=CARTESIAN_POINT('',(30.4914971157456,1.8,8.34350288425444));
#16762=CARTESIAN_POINT('',(30.4914971157456,-1.9,8.34350288425444));
#16763=CARTESIAN_POINT('Origin',(30.6564971157456,1.8,8.34350288425444));
#16764=CARTESIAN_POINT('Origin',(33.3435028842544,-1.9,8.34350288425444));
#16765=CARTESIAN_POINT('',(33.1785028842544,-1.8,8.34350288425444));
#16766=CARTESIAN_POINT('Origin',(33.3435028842544,-1.8,8.34350288425444));
#16767=CARTESIAN_POINT('',(33.1785028842544,1.8,8.34350288425444));
#16768=CARTESIAN_POINT('',(33.1785028842544,-1.9,8.34350288425444));
#16769=CARTESIAN_POINT('Origin',(33.3435028842544,1.8,8.34350288425444));
#16770=CARTESIAN_POINT('Origin',(33.3435028842544,-1.9,5.65649711574556));
#16771=CARTESIAN_POINT('',(33.1785028842544,-1.8,5.65649711574556));
#16772=CARTESIAN_POINT('Origin',(33.3435028842544,-1.8,5.65649711574556));
#16773=CARTESIAN_POINT('',(33.1785028842544,1.8,5.65649711574556));
#16774=CARTESIAN_POINT('',(33.1785028842544,-1.9,5.65649711574556));
#16775=CARTESIAN_POINT('Origin',(33.3435028842544,1.8,5.65649711574556));
#16776=CARTESIAN_POINT('Origin',(32.,-1.9,7.));
#16777=CARTESIAN_POINT('',(30.5,-1.8,7.));
#16778=CARTESIAN_POINT('Origin',(32.,-1.8,7.));
#16779=CARTESIAN_POINT('',(30.5,1.8,7.));
#16780=CARTESIAN_POINT('',(30.5,-1.9,7.));
#16781=CARTESIAN_POINT('Origin',(32.,1.8,7.));
#16782=CARTESIAN_POINT('Origin',(34.8,-1.,-0.1));
#16783=CARTESIAN_POINT('',(34.575,-1.,0.));
#16784=CARTESIAN_POINT('Origin',(34.8,-1.,0.));
#16785=CARTESIAN_POINT('',(34.575,-1.,0.8));
#16786=CARTESIAN_POINT('',(34.575,-1.,-0.1));
#16787=CARTESIAN_POINT('Origin',(34.8,-1.,0.8));
#16788=CARTESIAN_POINT('Origin',(29.2,1.,-0.1));
#16789=CARTESIAN_POINT('',(28.975,1.,0.));
#16790=CARTESIAN_POINT('Origin',(29.2,1.,0.));
#16791=CARTESIAN_POINT('',(28.975,1.,0.8));
#16792=CARTESIAN_POINT('',(28.975,1.,-0.1));
#16793=CARTESIAN_POINT('Origin',(29.2,1.,0.8));
#16794=CARTESIAN_POINT('Origin',(29.2,-1.,-0.1));
#16795=CARTESIAN_POINT('',(28.975,-1.,0.));
#16796=CARTESIAN_POINT('Origin',(29.2,-1.,0.));
#16797=CARTESIAN_POINT('',(28.975,-1.,0.8));
#16798=CARTESIAN_POINT('',(28.975,-1.,-0.1));
#16799=CARTESIAN_POINT('Origin',(29.2,-1.,0.8));
#16800=CARTESIAN_POINT('Origin',(34.8,1.,-0.1));
#16801=CARTESIAN_POINT('',(34.575,1.,0.));
#16802=CARTESIAN_POINT('Origin',(34.8,1.,0.));
#16803=CARTESIAN_POINT('',(34.575,1.,0.8));
#16804=CARTESIAN_POINT('',(34.575,1.,-0.1));
#16805=CARTESIAN_POINT('Origin',(34.8,1.,0.8));
#16806=CARTESIAN_POINT('Origin',(28.6,-1.8,0.8));
#16807=CARTESIAN_POINT('',(34.2,-1.8,0.8));
#16808=CARTESIAN_POINT('',(34.2,1.8,0.8));
#16809=CARTESIAN_POINT('',(34.2,-1.8,0.8));
#16810=CARTESIAN_POINT('',(35.4,-1.8,0.8));
#16811=CARTESIAN_POINT('',(35.4,-1.8,0.8));
#16812=CARTESIAN_POINT('',(35.4,1.8,0.8));
#16813=CARTESIAN_POINT('',(35.4,-1.8,0.8));
#16814=CARTESIAN_POINT('',(35.4,1.8,0.8));
#16815=CARTESIAN_POINT('Origin',(28.6,-1.8,0.8));
#16816=CARTESIAN_POINT('',(29.8,1.8,0.8));
#16817=CARTESIAN_POINT('',(29.8,-1.8,0.8));
#16818=CARTESIAN_POINT('',(29.8,0.,0.8));
#16819=CARTESIAN_POINT('',(28.6,1.8,0.8));
#16820=CARTESIAN_POINT('',(35.4,1.8,0.8));
#16821=CARTESIAN_POINT('',(28.6,-1.8,0.8));
#16822=CARTESIAN_POINT('',(28.6,-1.8,0.8));
#16823=CARTESIAN_POINT('',(35.4,-1.8,0.8));
#16824=CARTESIAN_POINT('Origin',(28.6,-1.8,0.));
#16825=CARTESIAN_POINT('',(28.6,-1.8,0.));
#16826=CARTESIAN_POINT('',(28.6,-1.8,0.8));
#16827=CARTESIAN_POINT('',(28.6,1.8,0.));
#16828=CARTESIAN_POINT('',(28.6,1.8,0.8));
#16829=CARTESIAN_POINT('',(28.6,-1.8,0.));
#16830=CARTESIAN_POINT('Origin',(35.4,-1.8,0.8));
#16831=CARTESIAN_POINT('',(35.4,-1.8,0.));
#16832=CARTESIAN_POINT('',(35.4,-1.8,0.));
#16833=CARTESIAN_POINT('',(35.4,1.8,0.));
#16834=CARTESIAN_POINT('',(35.4,-1.8,0.));
#16835=CARTESIAN_POINT('',(35.4,1.8,0.));
#16836=CARTESIAN_POINT('Origin',(29.8,-1.8,0.));
#16837=CARTESIAN_POINT('',(34.2,-1.8,9.2));
#16838=CARTESIAN_POINT('',(34.2,-1.8,0.));
#16839=CARTESIAN_POINT('',(29.8,-1.8,9.2));
#16840=CARTESIAN_POINT('',(29.8,-1.8,9.2));
#16841=CARTESIAN_POINT('',(29.8,-1.8,0.));
#16842=CARTESIAN_POINT('',(28.6,-1.8,0.));
#16843=CARTESIAN_POINT('Origin',(34.2,-1.8,0.));
#16844=CARTESIAN_POINT('',(34.2,1.8,9.2));
#16845=CARTESIAN_POINT('',(34.2,1.8,0.));
#16846=CARTESIAN_POINT('',(34.2,-1.8,9.2));
#16847=CARTESIAN_POINT('Origin',(34.2,1.8,0.));
#16848=CARTESIAN_POINT('',(29.8,1.8,9.2));
#16849=CARTESIAN_POINT('',(29.8,1.8,0.));
#16850=CARTESIAN_POINT('',(34.2,1.8,9.2));
#16851=CARTESIAN_POINT('',(28.6,1.8,0.));
#16852=CARTESIAN_POINT('Origin',(29.8,1.8,0.));
#16853=CARTESIAN_POINT('',(29.8,1.8,9.2));
#16854=CARTESIAN_POINT('Origin',(32.,0.,9.2));
#16855=CARTESIAN_POINT('Origin',(32.,0.,0.));
#19998=UNCERTAINTY_MEASURE_WITH_UNIT(LENGTH_MEASURE(0.001),#20097,
'DISTANCE_ACCURACY_VALUE',
'Maximum model space distance between geometric entities at asserted c
onnectivities');
#20042=UNCERTAINTY_MEASURE_WITH_UNIT(LENGTH_MEASURE(0.001),#20097,
'DISTANCE_ACCURACY_VALUE',
'Maximum model space distance between geometric entities at asserted c
onnectivities');
#20052=(
GEOMETRIC_REPRESENTATION_CONTEXT(3)
GLOBAL_UNCERTAINTY_ASSIGNED_CONTEXT((#19998))
GLOBAL_UNIT_ASSIGNED_CONTEXT((#20097,#20099,#20100))
REPRESENTATION_CONTEXT('','3D')
);
#20096=(
GEOMETRIC_REPRESENTATION_CONTEXT(3)
GLOBAL_UNCERTAINTY_ASSIGNED_CONTEXT((#20042))
GLOBAL_UNIT_ASSIGNED_CONTEXT((#20097,#20099,#20100))
REPRESENTATION_CONTEXT('','3D')
);
#20097=(
LENGTH_UNIT()
NAMED_UNIT(*)
SI_UNIT(.CENTI.,.METRE.)
);
#20099=(
NAMED_UNIT(*)
PLANE_ANGLE_UNIT()
SI_UNIT($,.RADIAN.)
);
#20100=(
NAMED_UNIT(*)
SI_UNIT($,.STERADIAN.)
SOLID_ANGLE_UNIT()
);
#20110=SHAPE_DEFINITION_REPRESENTATION(#20163,#20321);
#20163=PRODUCT_DEFINITION_SHAPE('',$,#20375);
#20321=SHAPE_REPRESENTATION('',(#11716),#20052);
#20365=PRODUCT_DEFINITION_CONTEXT('part definition',#20526,'design');
#20375=PRODUCT_DEFINITION('Fixed bearing block (1)',
'Fixed bearing block (1)',#20428,#20365);
#20428=PRODUCT_DEFINITION_FORMATION('',$,#20537);
#20526=APPLICATION_CONTEXT(
'Core Data for Automotive Mechanical Design Process');
#20527=PRODUCT_CONTEXT('part definition',#20526,'mechanical');
#20537=PRODUCT('Fixed bearing block (1)','Fixed bearing block (1)',
'Fixed bearing block (1)',(#20527));
#20644=COLOUR_RGB('Grey',0.48,0.52,0.57);
#20645=FILL_AREA_STYLE_COLOUR('',#20644);
#20646=FILL_AREA_STYLE('',(#20645));
#20647=SURFACE_STYLE_FILL_AREA(#20646);
#20648=SURFACE_SIDE_STYLE('',(#20647));
#20649=SURFACE_STYLE_USAGE(.BOTH.,#20648);
#20650=PRESENTATION_STYLE_ASSIGNMENT((#20649));
ENDSEC;
END-ISO-10303-21;
